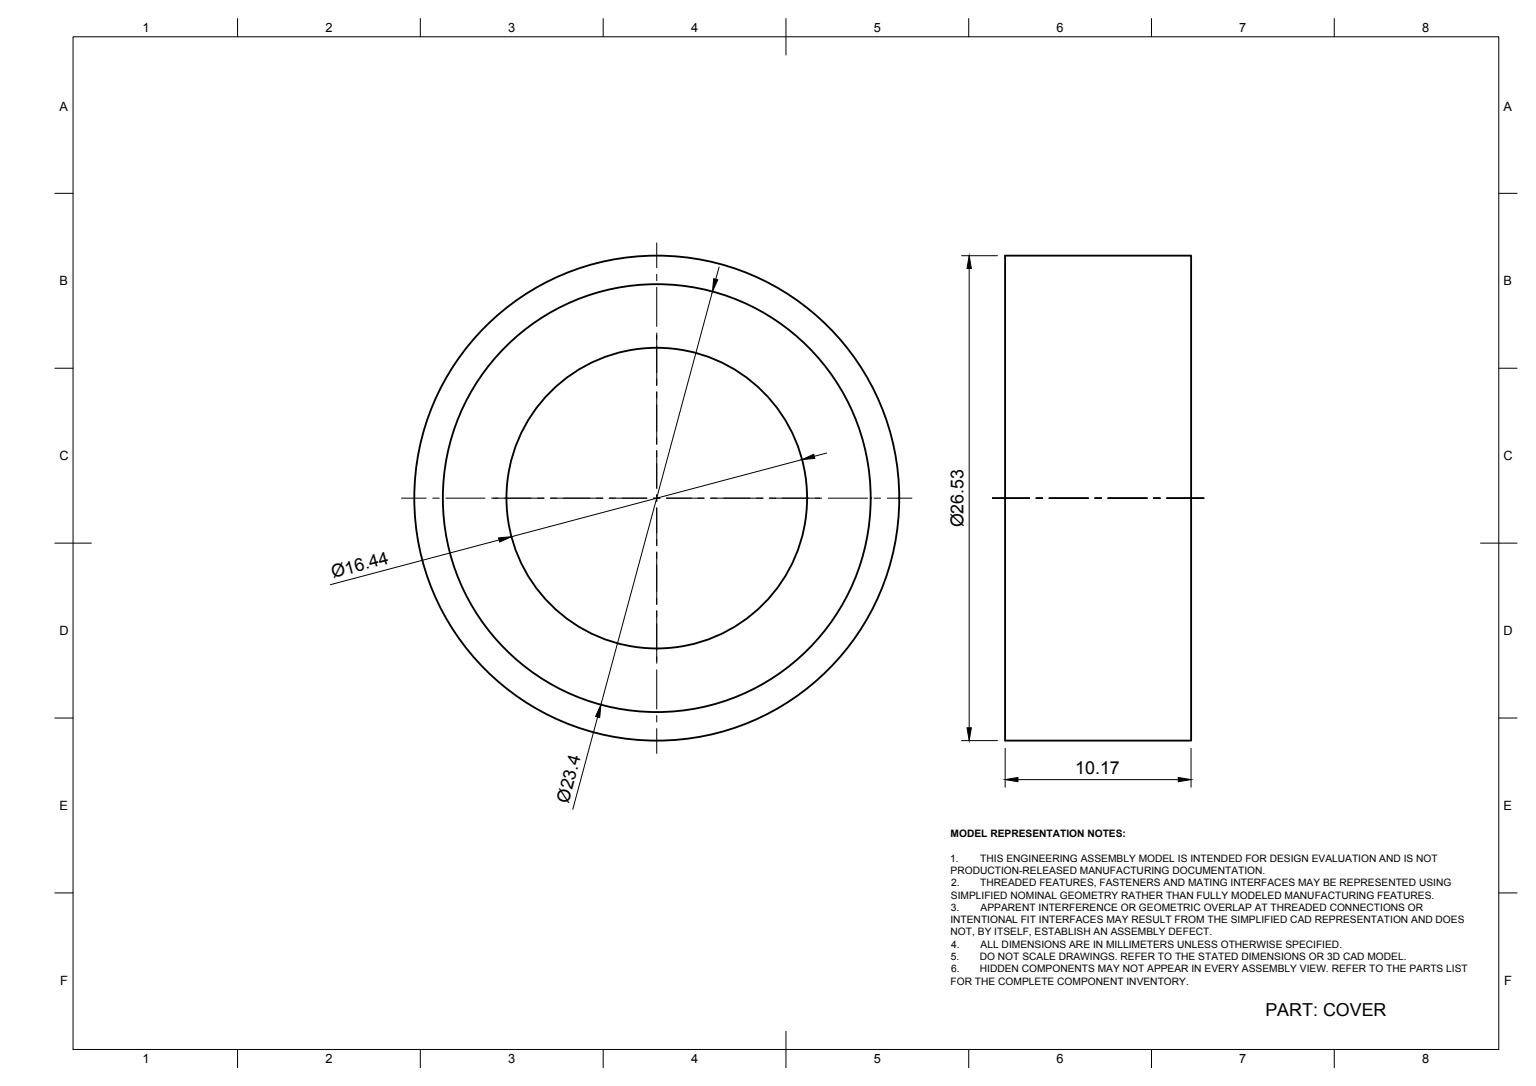
ISO-10303-21;
HEADER;
/* Generated by software containing ST-Developer
 * from STEP Tools, Inc. (www.steptools.com) 
 */

FILE_DESCRIPTION(
/* description */ (''),
/* implementation_level */ '2;1');

FILE_NAME(
/* name */ 'Cover.step',
/* time_stamp */ '2026-10-04T22:56:18-07:00',
/* author */ (''),
/* organization */ (''),
/* preprocessor_version */ 'ST-DEVELOPER v20.2',
/* originating_system */ 'Autodesk Translation Framework v15.15.0.0',
/* authorisation */ '');

FILE_SCHEMA (('AUTOMOTIVE_DESIGN { 1 0 10303 214 3 1 1 }'));
ENDSEC;

DATA;
#10=MECHANICAL_DESIGN_GEOMETRIC_PRESENTATION_REPRESENTATION('',(#194),#14544);
#178=SHAPE_REPRESENTATION_RELATIONSHIP('SRR','None',#14580,#186);
#186=ADVANCED_BREP_SHAPE_REPRESENTATION('',(#202),#14540);
#194=STYLED_ITEM('',(#14626),#202);
#202=MANIFOLD_SOLID_BREP('Body1',#1830);
#220=LINE('',#2712,#276);
#221=LINE('',#2720,#277);
#222=LINE('',#2727,#278);
#276=VECTOR('',#2284,8.2210249646156);
#277=VECTOR('',#2295,13.263882223741);
#278=VECTOR('',#2304,11.7021025234003);
#332=CYLINDRICAL_SURFACE('',#1992,8.2210249646156);
#333=CYLINDRICAL_SURFACE('',#1997,13.263882223741);
#334=CYLINDRICAL_SURFACE('',#2001,11.7021025234003);
#382=FACE_BOUND('',#549,.T.);
#383=FACE_BOUND('',#552,.T.);
#384=FACE_BOUND('',#555,.T.);
#430=FACE_OUTER_BOUND('',#547,.T.);
#431=FACE_OUTER_BOUND('',#548,.T.);
#432=FACE_OUTER_BOUND('',#550,.T.);
#433=FACE_OUTER_BOUND('',#551,.T.);
#434=FACE_OUTER_BOUND('',#553,.T.);
#435=FACE_OUTER_BOUND('',#554,.T.);
#547=EDGE_LOOP('',(#1263,#1264,#1265,#1266));
#548=EDGE_LOOP('',(#1267));
#549=EDGE_LOOP('',(#1268));
#550=EDGE_LOOP('',(#1269,#1270,#1271,#1272));
#551=EDGE_LOOP('',(#1273));
#552=EDGE_LOOP('',(#1274));
#553=EDGE_LOOP('',(#1275,#1276,#1277,#1278));
#554=EDGE_LOOP('',(#1279));
#555=EDGE_LOOP('',(#1280));
#670=CIRCLE('',#1993,8.2210249646156);
#671=CIRCLE('',#1994,8.2210249646156);
#672=CIRCLE('',#1996,13.263882223741);
#673=CIRCLE('',#1998,13.263882223741);
#674=CIRCLE('',#2000,11.7021025234003);
#675=CIRCLE('',#2002,11.7021025234003);
#756=VERTEX_POINT('',#2709);
#757=VERTEX_POINT('',#2711);
#758=VERTEX_POINT('',#2715);
#759=VERTEX_POINT('',#2718);
#760=VERTEX_POINT('',#2722);
#761=VERTEX_POINT('',#2725);
#960=EDGE_CURVE('',#756,#756,#670,.T.);
#961=EDGE_CURVE('',#756,#757,#220,.T.);
#962=EDGE_CURVE('',#757,#757,#671,.T.);
#963=EDGE_CURVE('',#758,#758,#672,.T.);
#964=EDGE_CURVE('',#759,#759,#673,.T.);
#965=EDGE_CURVE('',#759,#758,#221,.T.);
#966=EDGE_CURVE('',#760,#760,#674,.T.);
#967=EDGE_CURVE('',#761,#761,#675,.T.);
#968=EDGE_CURVE('',#761,#760,#222,.T.);
#1263=ORIENTED_EDGE('',*,*,#960,.F.);
#1264=ORIENTED_EDGE('',*,*,#961,.T.);
#1265=ORIENTED_EDGE('',*,*,#962,.T.);
#1266=ORIENTED_EDGE('',*,*,#961,.F.);
#1267=ORIENTED_EDGE('',*,*,#963,.F.);
#1268=ORIENTED_EDGE('',*,*,#960,.T.);
#1269=ORIENTED_EDGE('',*,*,#964,.F.);
#1270=ORIENTED_EDGE('',*,*,#965,.T.);
#1271=ORIENTED_EDGE('',*,*,#963,.T.);
#1272=ORIENTED_EDGE('',*,*,#965,.F.);
#1273=ORIENTED_EDGE('',*,*,#964,.T.);
#1274=ORIENTED_EDGE('',*,*,#966,.F.);
#1275=ORIENTED_EDGE('',*,*,#967,.F.);
#1276=ORIENTED_EDGE('',*,*,#968,.T.);
#1277=ORIENTED_EDGE('',*,*,#966,.T.);
#1278=ORIENTED_EDGE('',*,*,#968,.F.);
#1279=ORIENTED_EDGE('',*,*,#967,.T.);
#1280=ORIENTED_EDGE('',*,*,#962,.F.);
#1699=PLANE('',#1995);
#1700=PLANE('',#1999);
#1701=PLANE('',#2003);
#1752=ADVANCED_FACE('',(#430),#332,.F.);
#1753=ADVANCED_FACE('',(#431,#382),#1699,.T.);
#1754=ADVANCED_FACE('',(#432),#333,.T.);
#1755=ADVANCED_FACE('',(#433,#383),#1700,.T.);
#1756=ADVANCED_FACE('',(#434),#334,.F.);
#1757=ADVANCED_FACE('',(#435,#384),#1701,.T.);
#1830=CLOSED_SHELL('',(#1752,#1753,#1754,#1755,#1756,#1757));
#1991=AXIS2_PLACEMENT_3D('',#2707,#2278,#2279);
#1992=AXIS2_PLACEMENT_3D('',#2708,#2280,#2281);
#1993=AXIS2_PLACEMENT_3D('',#2710,#2282,#2283);
#1994=AXIS2_PLACEMENT_3D('',#2713,#2285,#2286);
#1995=AXIS2_PLACEMENT_3D('',#2714,#2287,#2288);
#1996=AXIS2_PLACEMENT_3D('',#2716,#2289,#2290);
#1997=AXIS2_PLACEMENT_3D('',#2717,#2291,#2292);
#1998=AXIS2_PLACEMENT_3D('',#2719,#2293,#2294);
#1999=AXIS2_PLACEMENT_3D('',#2721,#2296,#2297);
#2000=AXIS2_PLACEMENT_3D('',#2723,#2298,#2299);
#2001=AXIS2_PLACEMENT_3D('',#2724,#2300,#2301);
#2002=AXIS2_PLACEMENT_3D('',#2726,#2302,#2303);
#2003=AXIS2_PLACEMENT_3D('',#2728,#2305,#2306);
#2278=DIRECTION('axis',(0.,0.,1.));
#2279=DIRECTION('refdir',(1.,0.,0.));
#2280=DIRECTION('center_axis',(0.,0.,1.));
#2281=DIRECTION('ref_axis',(1.,0.,0.));
#2282=DIRECTION('center_axis',(0.,0.,1.));
#2283=DIRECTION('ref_axis',(1.,0.,0.));
#2284=DIRECTION('',(0.,0.,1.));
#2285=DIRECTION('center_axis',(0.,0.,1.));
#2286=DIRECTION('ref_axis',(1.,0.,0.));
#2287=DIRECTION('center_axis',(0.,0.,-1.));
#2288=DIRECTION('ref_axis',(-1.,0.,0.));
#2289=DIRECTION('center_axis',(0.,0.,1.));
#2290=DIRECTION('ref_axis',(1.,0.,0.));
#2291=DIRECTION('center_axis',(0.,0.,1.));
#2292=DIRECTION('ref_axis',(1.,0.,0.));
#2293=DIRECTION('center_axis',(0.,0.,1.));
#2294=DIRECTION('ref_axis',(1.,0.,0.));
#2295=DIRECTION('',(0.,0.,-1.));
#2296=DIRECTION('center_axis',(0.,0.,1.));
#2297=DIRECTION('ref_axis',(1.,0.,0.));
#2298=DIRECTION('center_axis',(0.,0.,1.));
#2299=DIRECTION('ref_axis',(1.,0.,0.));
#2300=DIRECTION('center_axis',(0.,0.,1.));
#2301=DIRECTION('ref_axis',(1.,0.,0.));
#2302=DIRECTION('center_axis',(0.,0.,1.));
#2303=DIRECTION('ref_axis',(1.,0.,0.));
#2304=DIRECTION('',(0.,0.,1.));
#2305=DIRECTION('center_axis',(0.,0.,1.));
#2306=DIRECTION('ref_axis',(1.,0.,0.));
#2707=CARTESIAN_POINT('',(0.,0.,0.));
#2708=CARTESIAN_POINT('Origin',(0.,0.,27.4843056886915));
#2709=CARTESIAN_POINT('',(-8.2210249646156,-1.0067851908627E-15,26.6343056886915));
#2710=CARTESIAN_POINT('Origin',(0.,0.,26.6343056886915));
#2711=CARTESIAN_POINT('',(-8.2210249646156,-1.0067851908627E-15,28.3343056886915));
#2712=CARTESIAN_POINT('',(-8.2210249646156,-1.0067851908627E-15,27.4843056886915));
#2713=CARTESIAN_POINT('Origin',(0.,0.,28.3343056886915));
#2714=CARTESIAN_POINT('Origin',(13.263882223741,0.,26.6343056886915));
#2715=CARTESIAN_POINT('',(-13.263882223741,-1.62435709095719E-15,26.6343056886915));
#2716=CARTESIAN_POINT('Origin',(0.,0.,26.6343056886915));
#2717=CARTESIAN_POINT('Origin',(0.,0.,31.7196089913165));
#2718=CARTESIAN_POINT('',(-13.263882223741,-1.62435709095719E-15,36.8049122939414));
#2719=CARTESIAN_POINT('Origin',(0.,0.,36.8049122939414));
#2720=CARTESIAN_POINT('',(-13.263882223741,-1.62435709095719E-15,31.7196089913165));
#2721=CARTESIAN_POINT('Origin',(11.7021025234003,0.,36.8049122939414));
#2722=CARTESIAN_POINT('',(-11.7021025234003,-1.43309423985764E-15,36.8049122939414));
#2723=CARTESIAN_POINT('Origin',(0.,0.,36.8049122939414));
#2724=CARTESIAN_POINT('Origin',(0.,0.,32.5696089913164));
#2725=CARTESIAN_POINT('',(-11.7021025234003,-1.43309423985764E-15,28.3343056886915));
#2726=CARTESIAN_POINT('Origin',(0.,0.,28.3343056886915));
#2727=CARTESIAN_POINT('',(-11.7021025234003,-1.43309423985763E-15,32.5696089913164));
#2728=CARTESIAN_POINT('Origin',(8.2210249646156,0.,28.3343056886915));
#14530=UNCERTAINTY_MEASURE_WITH_UNIT(LENGTH_MEASURE(0.01),#14545,
'DISTANCE_ACCURACY_VALUE',
'Maximum model space distance between geometric entities at asserted c
onnectivities');
#14534=UNCERTAINTY_MEASURE_WITH_UNIT(LENGTH_MEASURE(0.01),#14545,
'DISTANCE_ACCURACY_VALUE',
'Maximum model space distance between geometric entities at asserted c
onnectivities');
#14540=(
GEOMETRIC_REPRESENTATION_CONTEXT(3)
GLOBAL_UNCERTAINTY_ASSIGNED_CONTEXT((#14530))
GLOBAL_UNIT_ASSIGNED_CONTEXT((#14545,#14547,#14548))
REPRESENTATION_CONTEXT('','3D')
);
#14544=(
GEOMETRIC_REPRESENTATION_CONTEXT(3)
GLOBAL_UNCERTAINTY_ASSIGNED_CONTEXT((#14534))
GLOBAL_UNIT_ASSIGNED_CONTEXT((#14545,#14547,#14548))
REPRESENTATION_CONTEXT('','3D')
);
#14545=(
LENGTH_UNIT()
NAMED_UNIT(*)
SI_UNIT(.MILLI.,.METRE.)
);
#14547=(
NAMED_UNIT(*)
PLANE_ANGLE_UNIT()
SI_UNIT($,.RADIAN.)
);
#14548=(
NAMED_UNIT(*)
SI_UNIT($,.STERADIAN.)
SOLID_ANGLE_UNIT()
);
#14554=SHAPE_DEFINITION_REPRESENTATION(#14563,#14580);
#14563=PRODUCT_DEFINITION_SHAPE('',$,#14590);
#14580=SHAPE_REPRESENTATION('',(#1991),#14540);
#14584=PRODUCT_DEFINITION_CONTEXT('part definition',#14613,'design');
#14590=PRODUCT_DEFINITION('Cover','Cover',#14599,#14584);
#14599=PRODUCT_DEFINITION_FORMATION('',$,#14620);
#14613=APPLICATION_CONTEXT(
'Core Data for Automotive Mechanical Design Process');
#14614=PRODUCT_CONTEXT('part definition',#14613,'mechanical');
#14620=PRODUCT('Cover','Cover',$,(#14614));
#14626=PRESENTATION_STYLE_ASSIGNMENT((#14630));
#14630=SURFACE_STYLE_USAGE(.BOTH.,#14634);
#14634=SURFACE_SIDE_STYLE('',(#14638));
#14638=SURFACE_STYLE_FILL_AREA(#14642);
#14642=FILL_AREA_STYLE('Opaque(39,39,39)',(#14646));
#14646=FILL_AREA_STYLE_COLOUR('Opaque(39,39,39)',#14650);
#14650=COLOUR_RGB('Opaque(39,39,39)', 0.66274510, 0.83137255, 0.94901961);
ENDSEC;
END-ISO-10303-21;
